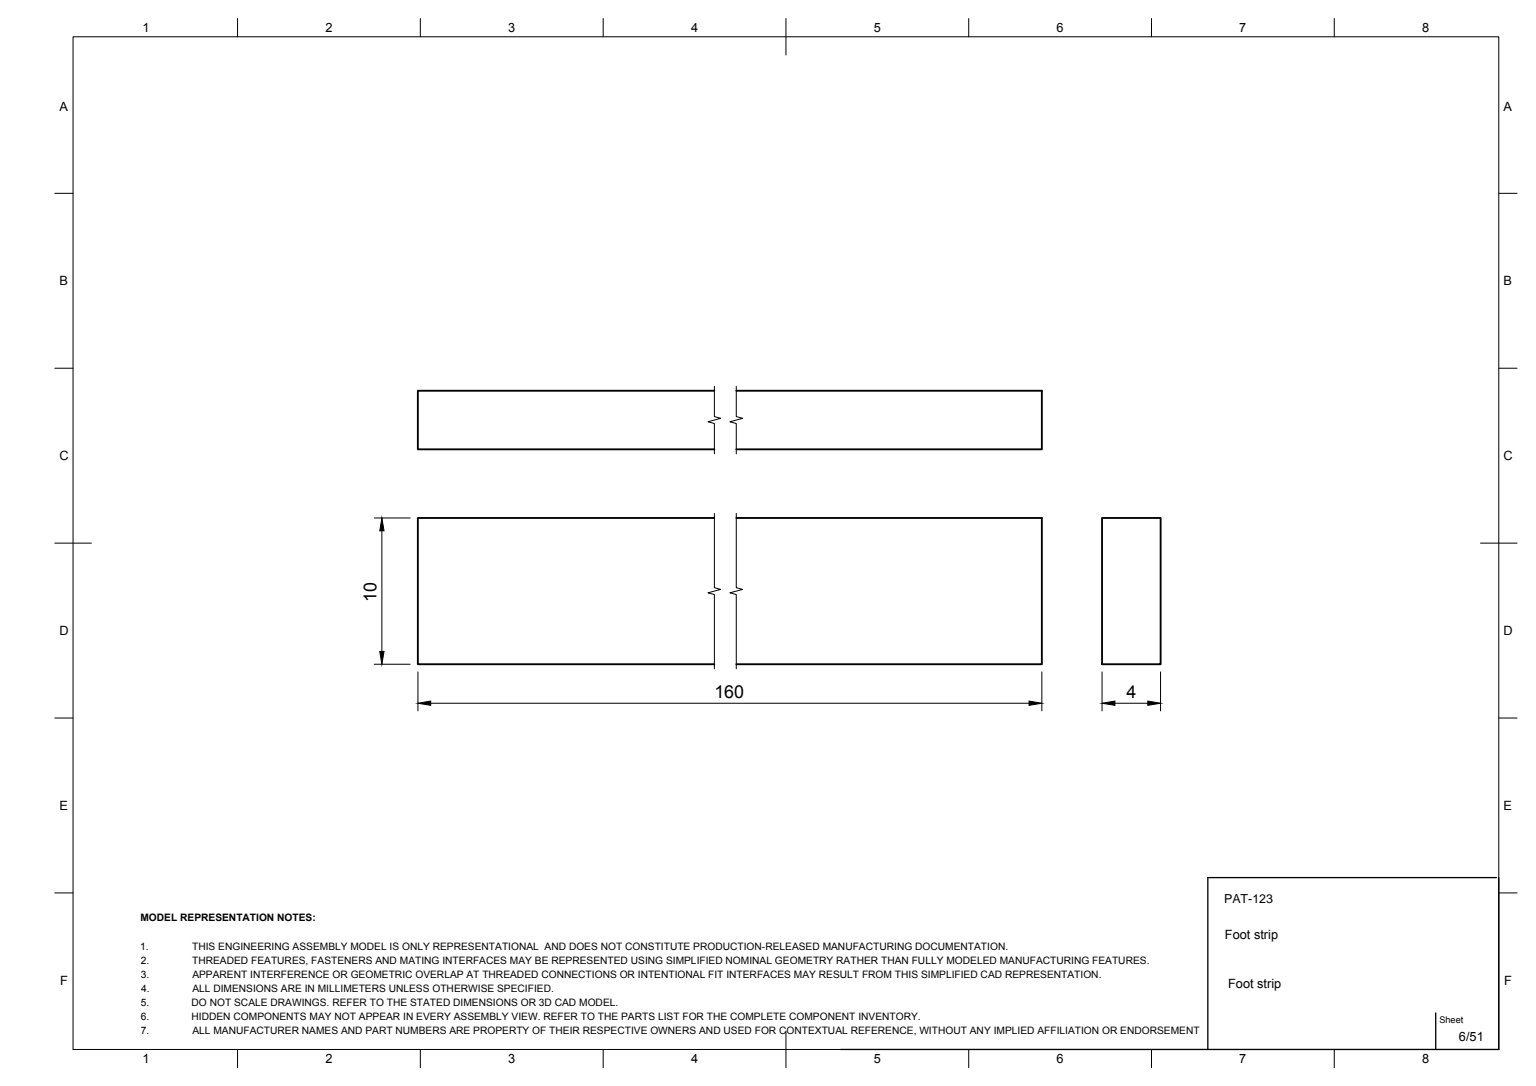
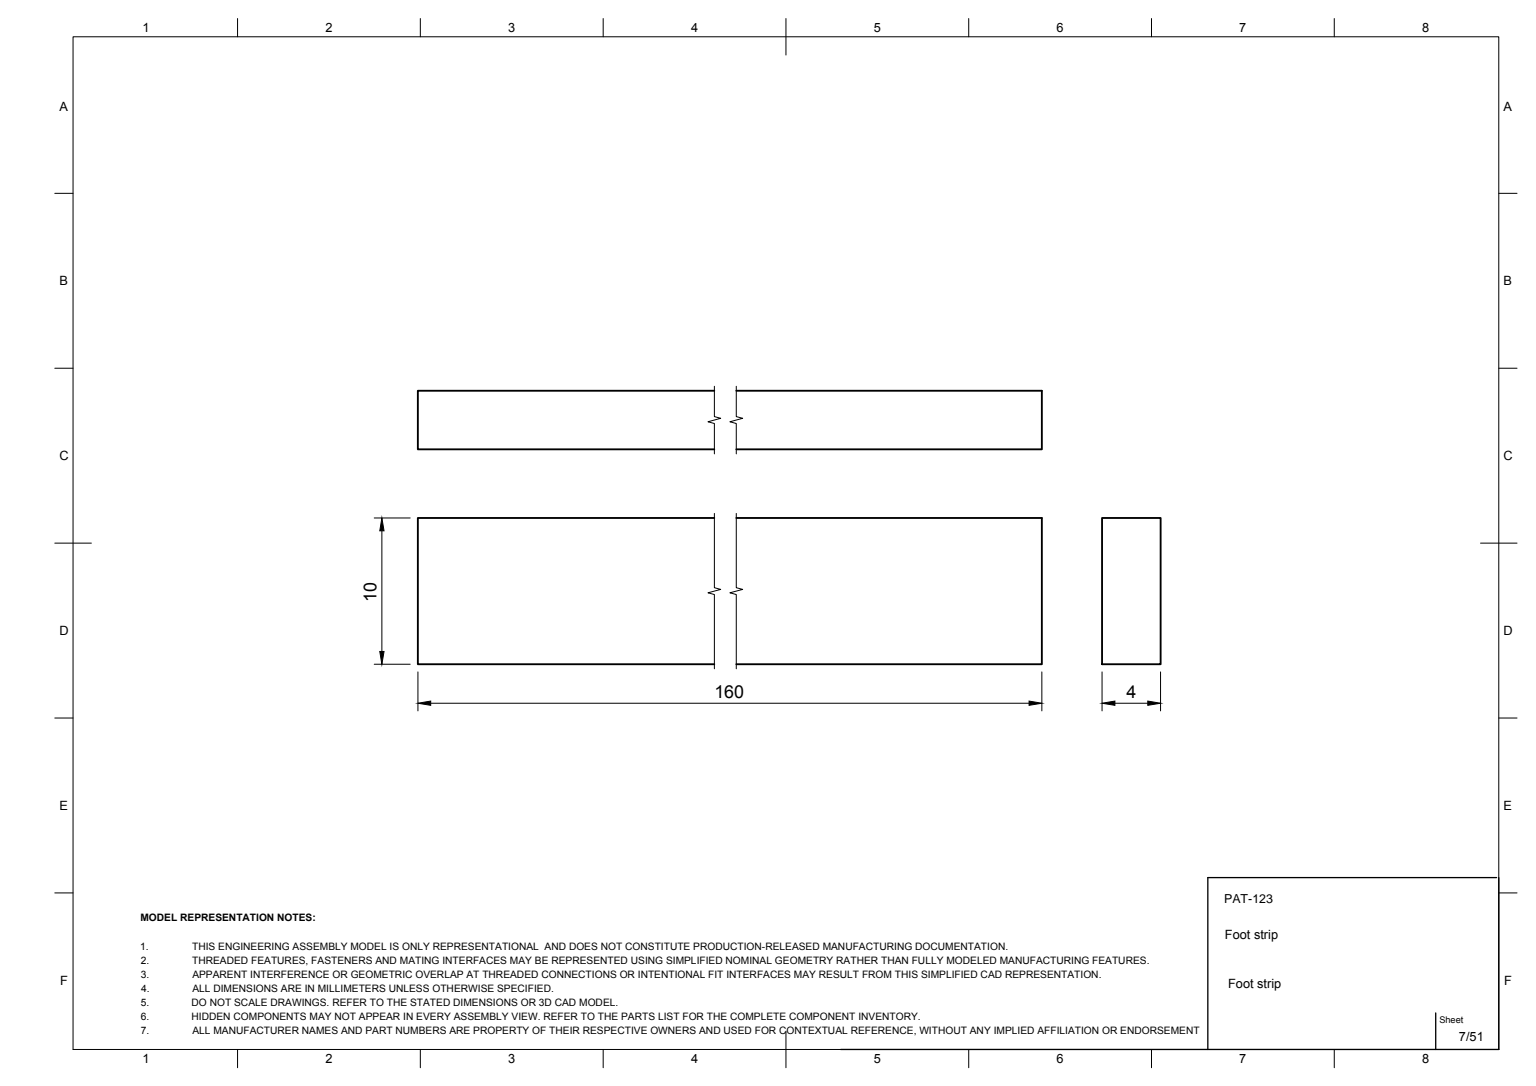
ISO-10303-21;
HEADER;
/* Generated by software containing ST-Developer
 * from STEP Tools, Inc. (www.steptools.com) 
 */

FILE_DESCRIPTION(
/* description */ ('Worm-less right-angle friction wheel drive'),
/* implementation_level */ '2;1');

FILE_NAME(
/* name */ 'Foot strip.step',
/* time_stamp */ '2026-10-28T03:22:36-07:00',
/* author */ (''),
/* organization */ (''),
/* preprocessor_version */ 'ST-DEVELOPER v20.2',
/* originating_system */ 'Autodesk Translation Framework v15.17.0.0',
/* authorisation */ '');

FILE_SCHEMA (('AUTOMOTIVE_DESIGN { 1 0 10303 214 3 1 1 }'));
ENDSEC;

DATA;
#10=MECHANICAL_DESIGN_GEOMETRIC_PRESENTATION_REPRESENTATION('',(#612),#17046);
#518=SHAPE_REPRESENTATION_RELATIONSHIP('SRR','None',#17261,#565);
#565=ADVANCED_BREP_SHAPE_REPRESENTATION('',(#666),#16997);
#612=STYLED_ITEM('',(#17577),#666);
#666=MANIFOLD_SOLID_BREP('Body1',#8167);
#958=PLANE('',#8782);
#959=PLANE('',#8783);
#960=PLANE('',#8784);
#961=PLANE('',#8785);
#962=PLANE('',#8786);
#963=PLANE('',#8787);
#1224=FACE_OUTER_BOUND('',#1710,.T.);
#1225=FACE_OUTER_BOUND('',#1711,.T.);
#1226=FACE_OUTER_BOUND('',#1712,.T.);
#1227=FACE_OUTER_BOUND('',#1713,.T.);
#1228=FACE_OUTER_BOUND('',#1714,.T.);
#1229=FACE_OUTER_BOUND('',#1715,.T.);
#1710=EDGE_LOOP('',(#5618,#5619,#5620,#5621));
#1711=EDGE_LOOP('',(#5622,#5623,#5624,#5625));
#1712=EDGE_LOOP('',(#5626,#5627,#5628,#5629));
#1713=EDGE_LOOP('',(#5630,#5631,#5632,#5633));
#1714=EDGE_LOOP('',(#5634,#5635,#5636,#5637));
#1715=EDGE_LOOP('',(#5638,#5639,#5640,#5641));
#2399=LINE('',#12468,#2939);
#2400=LINE('',#12470,#2940);
#2401=LINE('',#12472,#2941);
#2402=LINE('',#12473,#2942);
#2403=LINE('',#12476,#2943);
#2404=LINE('',#12478,#2944);
#2405=LINE('',#12479,#2945);
#2406=LINE('',#12482,#2946);
#2407=LINE('',#12484,#2947);
#2408=LINE('',#12485,#2948);
#2409=LINE('',#12487,#2949);
#2410=LINE('',#12488,#2950);
#2939=VECTOR('',#9877,1.);
#2940=VECTOR('',#9878,1.);
#2941=VECTOR('',#9879,1.);
#2942=VECTOR('',#9880,1.);
#2943=VECTOR('',#9883,1.);
#2944=VECTOR('',#9884,1.);
#2945=VECTOR('',#9885,1.);
#2946=VECTOR('',#9888,1.);
#2947=VECTOR('',#9889,1.);
#2948=VECTOR('',#9890,1.);
#2949=VECTOR('',#9893,1.);
#2950=VECTOR('',#9894,1.);
#3897=VERTEX_POINT('',#12466);
#3898=VERTEX_POINT('',#12467);
#3899=VERTEX_POINT('',#12469);
#3900=VERTEX_POINT('',#12471);
#3901=VERTEX_POINT('',#12475);
#3902=VERTEX_POINT('',#12477);
#3903=VERTEX_POINT('',#12481);
#3904=VERTEX_POINT('',#12483);
#4578=EDGE_CURVE('',#3897,#3898,#2399,.T.);
#4579=EDGE_CURVE('',#3898,#3899,#2400,.T.);
#4580=EDGE_CURVE('',#3900,#3899,#2401,.T.);
#4581=EDGE_CURVE('',#3897,#3900,#2402,.T.);
#4582=EDGE_CURVE('',#3901,#3897,#2403,.T.);
#4583=EDGE_CURVE('',#3902,#3900,#2404,.T.);
#4584=EDGE_CURVE('',#3901,#3902,#2405,.T.);
#4585=EDGE_CURVE('',#3903,#3901,#2406,.T.);
#4586=EDGE_CURVE('',#3904,#3902,#2407,.T.);
#4587=EDGE_CURVE('',#3903,#3904,#2408,.T.);
#4588=EDGE_CURVE('',#3898,#3903,#2409,.T.);
#4589=EDGE_CURVE('',#3899,#3904,#2410,.T.);
#5618=ORIENTED_EDGE('',*,*,#4578,.T.);
#5619=ORIENTED_EDGE('',*,*,#4579,.T.);
#5620=ORIENTED_EDGE('',*,*,#4580,.F.);
#5621=ORIENTED_EDGE('',*,*,#4581,.F.);
#5622=ORIENTED_EDGE('',*,*,#4582,.T.);
#5623=ORIENTED_EDGE('',*,*,#4581,.T.);
#5624=ORIENTED_EDGE('',*,*,#4583,.F.);
#5625=ORIENTED_EDGE('',*,*,#4584,.F.);
#5626=ORIENTED_EDGE('',*,*,#4585,.T.);
#5627=ORIENTED_EDGE('',*,*,#4584,.T.);
#5628=ORIENTED_EDGE('',*,*,#4586,.F.);
#5629=ORIENTED_EDGE('',*,*,#4587,.F.);
#5630=ORIENTED_EDGE('',*,*,#4588,.T.);
#5631=ORIENTED_EDGE('',*,*,#4587,.T.);
#5632=ORIENTED_EDGE('',*,*,#4589,.F.);
#5633=ORIENTED_EDGE('',*,*,#4579,.F.);
#5634=ORIENTED_EDGE('',*,*,#4589,.T.);
#5635=ORIENTED_EDGE('',*,*,#4586,.T.);
#5636=ORIENTED_EDGE('',*,*,#4583,.T.);
#5637=ORIENTED_EDGE('',*,*,#4580,.T.);
#5638=ORIENTED_EDGE('',*,*,#4588,.F.);
#5639=ORIENTED_EDGE('',*,*,#4578,.F.);
#5640=ORIENTED_EDGE('',*,*,#4582,.F.);
#5641=ORIENTED_EDGE('',*,*,#4585,.F.);
#7716=ADVANCED_FACE('',(#1224),#958,.T.);
#7717=ADVANCED_FACE('',(#1225),#959,.T.);
#7718=ADVANCED_FACE('',(#1226),#960,.T.);
#7719=ADVANCED_FACE('',(#1227),#961,.T.);
#7720=ADVANCED_FACE('',(#1228),#962,.T.);
#7721=ADVANCED_FACE('',(#1229),#963,.F.);
#8167=CLOSED_SHELL('',(#7716,#7717,#7718,#7719,#7720,#7721));
#8781=AXIS2_PLACEMENT_3D('',#12464,#9873,#9874);
#8782=AXIS2_PLACEMENT_3D('',#12465,#9875,#9876);
#8783=AXIS2_PLACEMENT_3D('',#12474,#9881,#9882);
#8784=AXIS2_PLACEMENT_3D('',#12480,#9886,#9887);
#8785=AXIS2_PLACEMENT_3D('',#12486,#9891,#9892);
#8786=AXIS2_PLACEMENT_3D('',#12489,#9895,#9896);
#8787=AXIS2_PLACEMENT_3D('',#12490,#9897,#9898);
#9873=DIRECTION('axis',(0.,0.,1.));
#9874=DIRECTION('refdir',(1.,0.,0.));
#9875=DIRECTION('center_axis',(0.,1.,0.));
#9876=DIRECTION('ref_axis',(-1.,0.,0.));
#9877=DIRECTION('',(-1.,0.,0.));
#9878=DIRECTION('',(0.,0.,1.));
#9879=DIRECTION('',(-1.,0.,0.));
#9880=DIRECTION('',(0.,0.,1.));
#9881=DIRECTION('center_axis',(1.,0.,0.));
#9882=DIRECTION('ref_axis',(0.,1.,0.));
#9883=DIRECTION('',(0.,1.,0.));
#9884=DIRECTION('',(0.,1.,0.));
#9885=DIRECTION('',(0.,0.,1.));
#9886=DIRECTION('center_axis',(0.,-1.,0.));
#9887=DIRECTION('ref_axis',(1.,0.,0.));
#9888=DIRECTION('',(1.,0.,0.));
#9889=DIRECTION('',(1.,0.,0.));
#9890=DIRECTION('',(0.,0.,1.));
#9891=DIRECTION('center_axis',(-1.,0.,0.));
#9892=DIRECTION('ref_axis',(0.,-1.,0.));
#9893=DIRECTION('',(0.,-1.,0.));
#9894=DIRECTION('',(0.,-1.,0.));
#9895=DIRECTION('center_axis',(0.,0.,1.));
#9896=DIRECTION('ref_axis',(1.,0.,0.));
#9897=DIRECTION('center_axis',(0.,0.,1.));
#9898=DIRECTION('ref_axis',(1.,0.,0.));
#12464=CARTESIAN_POINT('',(0.,0.,0.));
#12465=CARTESIAN_POINT('Origin',(10.,-9.,-0.4));
#12466=CARTESIAN_POINT('',(10.,-9.,-0.4));
#12467=CARTESIAN_POINT('',(-6.,-9.,-0.4));
#12468=CARTESIAN_POINT('',(10.,-9.,-0.4));
#12469=CARTESIAN_POINT('',(-6.,-9.,0.));
#12470=CARTESIAN_POINT('',(-6.,-9.,-0.4));
#12471=CARTESIAN_POINT('',(10.,-9.,0.));
#12472=CARTESIAN_POINT('',(10.,-9.,0.));
#12473=CARTESIAN_POINT('',(10.,-9.,-0.4));
#12474=CARTESIAN_POINT('Origin',(10.,-10.,-0.4));
#12475=CARTESIAN_POINT('',(10.,-10.,-0.4));
#12476=CARTESIAN_POINT('',(10.,-10.,-0.4));
#12477=CARTESIAN_POINT('',(10.,-10.,0.));
#12478=CARTESIAN_POINT('',(10.,-10.,0.));
#12479=CARTESIAN_POINT('',(10.,-10.,-0.4));
#12480=CARTESIAN_POINT('Origin',(-6.,-10.,-0.4));
#12481=CARTESIAN_POINT('',(-6.,-10.,-0.4));
#12482=CARTESIAN_POINT('',(-6.,-10.,-0.4));
#12483=CARTESIAN_POINT('',(-6.,-10.,0.));
#12484=CARTESIAN_POINT('',(-6.,-10.,0.));
#12485=CARTESIAN_POINT('',(-6.,-10.,-0.4));
#12486=CARTESIAN_POINT('Origin',(-6.,-9.,-0.4));
#12487=CARTESIAN_POINT('',(-6.,-9.,-0.4));
#12488=CARTESIAN_POINT('',(-6.,-9.,0.));
#12489=CARTESIAN_POINT('Origin',(2.,-9.5,0.));
#12490=CARTESIAN_POINT('Origin',(2.,-9.5,-0.4));
#16944=UNCERTAINTY_MEASURE_WITH_UNIT(LENGTH_MEASURE(0.001),#17047,
'DISTANCE_ACCURACY_VALUE',
'Maximum model space distance between geometric entities at asserted c
onnectivities');
#16993=UNCERTAINTY_MEASURE_WITH_UNIT(LENGTH_MEASURE(0.001),#17047,
'DISTANCE_ACCURACY_VALUE',
'Maximum model space distance between geometric entities at asserted c
onnectivities');
#16997=(
GEOMETRIC_REPRESENTATION_CONTEXT(3)
GLOBAL_UNCERTAINTY_ASSIGNED_CONTEXT((#16944))
GLOBAL_UNIT_ASSIGNED_CONTEXT((#17047,#17049,#17050))
REPRESENTATION_CONTEXT('','3D')
);
#17046=(
GEOMETRIC_REPRESENTATION_CONTEXT(3)
GLOBAL_UNCERTAINTY_ASSIGNED_CONTEXT((#16993))
GLOBAL_UNIT_ASSIGNED_CONTEXT((#17047,#17049,#17050))
REPRESENTATION_CONTEXT('','3D')
);
#17047=(
LENGTH_UNIT()
NAMED_UNIT(*)
SI_UNIT(.CENTI.,.METRE.)
);
#17049=(
NAMED_UNIT(*)
PLANE_ANGLE_UNIT()
SI_UNIT($,.RADIAN.)
);
#17050=(
NAMED_UNIT(*)
SI_UNIT($,.STERADIAN.)
SOLID_ANGLE_UNIT()
);
#17054=SHAPE_DEFINITION_REPRESENTATION(#17106,#17261);
#17106=PRODUCT_DEFINITION_SHAPE('',$,#17314);
#17261=SHAPE_REPRESENTATION('',(#8781),#16997);
#17310=PRODUCT_DEFINITION_CONTEXT('part definition',#17468,'design');
#17314=PRODUCT_DEFINITION('Foot strip','Foot strip',#17366,#17310);
#17366=PRODUCT_DEFINITION_FORMATION('',$,#17473);
#17468=APPLICATION_CONTEXT(
'Core Data for Automotive Mechanical Design Process');
#17469=PRODUCT_CONTEXT('part definition',#17468,'mechanical');
#17473=PRODUCT('Foot strip','Foot strip','Foot strip',(#17469));
#17571=COLOUR_RGB('Light Blue',0.38,0.62,0.78);
#17572=FILL_AREA_STYLE_COLOUR('',#17571);
#17573=FILL_AREA_STYLE('',(#17572));
#17574=SURFACE_STYLE_FILL_AREA(#17573);
#17575=SURFACE_SIDE_STYLE('',(#17574));
#17576=SURFACE_STYLE_USAGE(.BOTH.,#17575);
#17577=PRESENTATION_STYLE_ASSIGNMENT((#17576));
ENDSEC;
END-ISO-10303-21;
